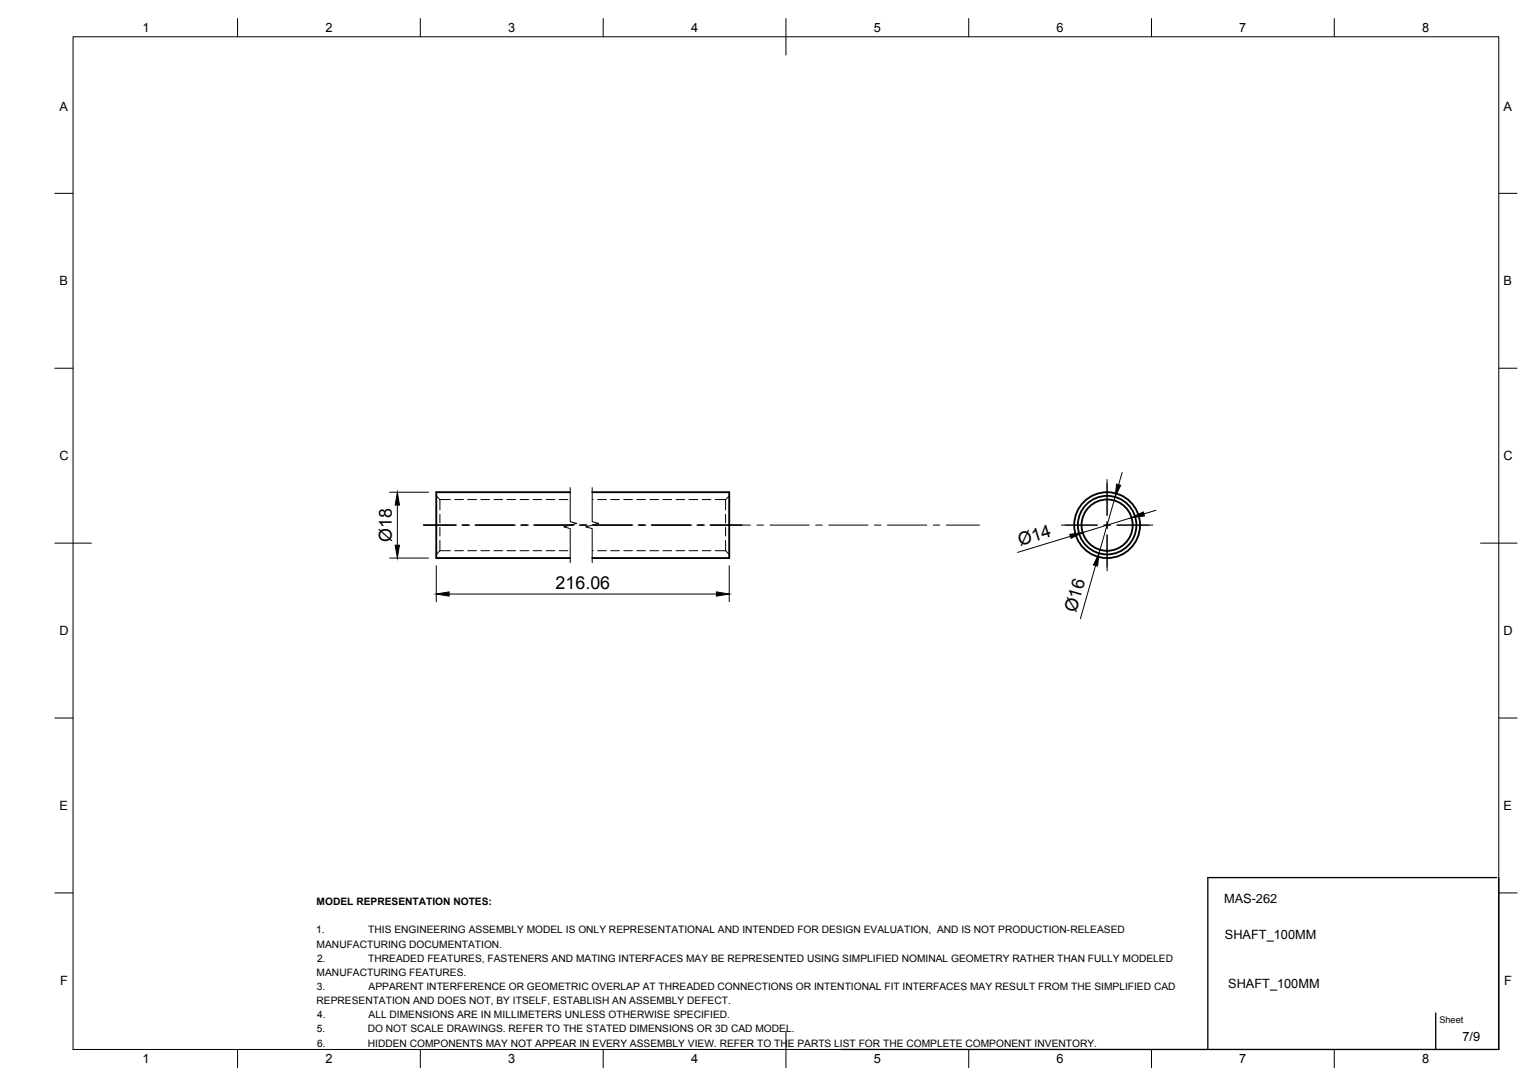
ISO-10303-21;
HEADER;
/* Generated by software containing ST-Developer
 * from STEP Tools, Inc. (www.steptools.com) 
 */

FILE_DESCRIPTION(
/* description */ (''),
/* implementation_level */ '2;1');

FILE_NAME(
/* name */ 'SHAFT_100MM.step',
/* time_stamp */ '2026-10-07T02:13:48+06:00',
/* author */ (''),
/* organization */ (''),
/* preprocessor_version */ 'ST-DEVELOPER v20.2',
/* originating_system */ 'Autodesk Translation Framework v15.15.0.0',
/* authorisation */ '');

FILE_SCHEMA (('AUTOMOTIVE_DESIGN { 1 0 10303 214 3 1 1 }'));
ENDSEC;

DATA;
#10=MECHANICAL_DESIGN_GEOMETRIC_PRESENTATION_REPRESENTATION('',(#118),#17042);
#59=CONICAL_SURFACE('',#8827,7.5,0.785398163397441);
#60=CONICAL_SURFACE('',#8834,7.5,0.785398163397441);
#94=SHAPE_REPRESENTATION_RELATIONSHIP('SRR','None',#17090,#106);
#106=ADVANCED_BREP_SHAPE_REPRESENTATION('',(#130),#17034);
#118=STYLED_ITEM('',(#17154),#130);
#130=MANIFOLD_SOLID_BREP('Body1',#8119);
#162=FACE_BOUND('',#1264,.T.);
#163=FACE_BOUND('',#1267,.T.);
#392=PLANE('',#8832);
#393=PLANE('',#8836);
#760=FACE_OUTER_BOUND('',#1261,.T.);
#761=FACE_OUTER_BOUND('',#1262,.T.);
#762=FACE_OUTER_BOUND('',#1263,.T.);
#763=FACE_OUTER_BOUND('',#1265,.T.);
#764=FACE_OUTER_BOUND('',#1266,.T.);
#765=FACE_OUTER_BOUND('',#1268,.T.);
#1261=EDGE_LOOP('',(#6519,#6520,#6521,#6522));
#1262=EDGE_LOOP('',(#6523,#6524,#6525,#6526));
#1263=EDGE_LOOP('',(#6527));
#1264=EDGE_LOOP('',(#6528));
#1265=EDGE_LOOP('',(#6529,#6530,#6531,#6532));
#1266=EDGE_LOOP('',(#6533));
#1267=EDGE_LOOP('',(#6534));
#1268=EDGE_LOOP('',(#6535,#6536,#6537,#6538));
#1764=CIRCLE('',#8828,8.);
#1765=CIRCLE('',#8829,7.);
#1766=CIRCLE('',#8831,7.);
#1767=CIRCLE('',#8833,9.);
#1768=CIRCLE('',#8835,8.);
#1769=CIRCLE('',#8837,9.);
#2426=LINE('',#13679,#3004);
#2427=LINE('',#13684,#3005);
#2428=LINE('',#13691,#3006);
#2429=LINE('',#13696,#3007);
#3004=VECTOR('',#10793,7.5);
#3005=VECTOR('',#10800,8.);
#3006=VECTOR('',#10809,7.5);
#3007=VECTOR('',#10816,9.);
#3619=VERTEX_POINT('',#13676);
#3620=VERTEX_POINT('',#13678);
#3621=VERTEX_POINT('',#13682);
#3622=VERTEX_POINT('',#13686);
#3623=VERTEX_POINT('',#13689);
#3624=VERTEX_POINT('',#13693);
#4627=EDGE_CURVE('',#3619,#3619,#1764,.T.);
#4628=EDGE_CURVE('',#3619,#3620,#2426,.T.);
#4629=EDGE_CURVE('',#3620,#3620,#1765,.T.);
#4630=EDGE_CURVE('',#3621,#3621,#1766,.T.);
#4631=EDGE_CURVE('',#3621,#3620,#2427,.T.);
#4632=EDGE_CURVE('',#3622,#3622,#1767,.T.);
#4633=EDGE_CURVE('',#3623,#3623,#1768,.T.);
#4634=EDGE_CURVE('',#3623,#3621,#2428,.T.);
#4635=EDGE_CURVE('',#3624,#3624,#1769,.T.);
#4636=EDGE_CURVE('',#3624,#3622,#2429,.T.);
#6519=ORIENTED_EDGE('',*,*,#4627,.T.);
#6520=ORIENTED_EDGE('',*,*,#4628,.T.);
#6521=ORIENTED_EDGE('',*,*,#4629,.T.);
#6522=ORIENTED_EDGE('',*,*,#4628,.F.);
#6523=ORIENTED_EDGE('',*,*,#4630,.F.);
#6524=ORIENTED_EDGE('',*,*,#4631,.T.);
#6525=ORIENTED_EDGE('',*,*,#4629,.F.);
#6526=ORIENTED_EDGE('',*,*,#4631,.F.);
#6527=ORIENTED_EDGE('',*,*,#4632,.T.);
#6528=ORIENTED_EDGE('',*,*,#4627,.F.);
#6529=ORIENTED_EDGE('',*,*,#4633,.T.);
#6530=ORIENTED_EDGE('',*,*,#4634,.T.);
#6531=ORIENTED_EDGE('',*,*,#4630,.T.);
#6532=ORIENTED_EDGE('',*,*,#4634,.F.);
#6533=ORIENTED_EDGE('',*,*,#4635,.T.);
#6534=ORIENTED_EDGE('',*,*,#4633,.F.);
#6535=ORIENTED_EDGE('',*,*,#4635,.F.);
#6536=ORIENTED_EDGE('',*,*,#4636,.T.);
#6537=ORIENTED_EDGE('',*,*,#4632,.F.);
#6538=ORIENTED_EDGE('',*,*,#4636,.F.);
#7569=CYLINDRICAL_SURFACE('',#8830,7.);
#7570=CYLINDRICAL_SURFACE('',#8838,9.);
#7922=ADVANCED_FACE('',(#760),#59,.F.);
#7923=ADVANCED_FACE('',(#761),#7569,.F.);
#7924=ADVANCED_FACE('',(#762,#162),#392,.T.);
#7925=ADVANCED_FACE('',(#763),#60,.F.);
#7926=ADVANCED_FACE('',(#764,#163),#393,.F.);
#7927=ADVANCED_FACE('',(#765),#7570,.T.);
#8119=CLOSED_SHELL('',(#7922,#7923,#7924,#7925,#7926,#7927));
#8826=AXIS2_PLACEMENT_3D('',#13674,#10787,#10788);
#8827=AXIS2_PLACEMENT_3D('',#13675,#10789,#10790);
#8828=AXIS2_PLACEMENT_3D('',#13677,#10791,#10792);
#8829=AXIS2_PLACEMENT_3D('',#13680,#10794,#10795);
#8830=AXIS2_PLACEMENT_3D('',#13681,#10796,#10797);
#8831=AXIS2_PLACEMENT_3D('',#13683,#10798,#10799);
#8832=AXIS2_PLACEMENT_3D('',#13685,#10801,#10802);
#8833=AXIS2_PLACEMENT_3D('',#13687,#10803,#10804);
#8834=AXIS2_PLACEMENT_3D('',#13688,#10805,#10806);
#8835=AXIS2_PLACEMENT_3D('',#13690,#10807,#10808);
#8836=AXIS2_PLACEMENT_3D('',#13692,#10810,#10811);
#8837=AXIS2_PLACEMENT_3D('',#13694,#10812,#10813);
#8838=AXIS2_PLACEMENT_3D('',#13695,#10814,#10815);
#10787=DIRECTION('axis',(0.,0.,1.));
#10788=DIRECTION('refdir',(1.,0.,0.));
#10789=DIRECTION('center_axis',(0.,0.,-1.));
#10790=DIRECTION('ref_axis',(-1.,0.,0.));
#10791=DIRECTION('center_axis',(0.,0.,-1.));
#10792=DIRECTION('ref_axis',(-1.,0.,0.));
#10793=DIRECTION('',(-0.707106781186542,8.65956056235487E-17,0.707106781186553));
#10794=DIRECTION('center_axis',(0.,0.,1.));
#10795=DIRECTION('ref_axis',(-1.,0.,0.));
#10796=DIRECTION('center_axis',(0.,0.,1.));
#10797=DIRECTION('ref_axis',(-1.,0.,0.));
#10798=DIRECTION('center_axis',(0.,0.,-1.));
#10799=DIRECTION('ref_axis',(-1.,0.,0.));
#10800=DIRECTION('',(0.,0.,-1.));
#10801=DIRECTION('center_axis',(0.,0.,-1.));
#10802=DIRECTION('ref_axis',(-1.,0.,0.));
#10803=DIRECTION('center_axis',(0.,0.,-1.));
#10804=DIRECTION('ref_axis',(-1.,0.,0.));
#10805=DIRECTION('center_axis',(0.,0.,1.));
#10806=DIRECTION('ref_axis',(-1.,0.,0.));
#10807=DIRECTION('center_axis',(0.,0.,1.));
#10808=DIRECTION('ref_axis',(-1.,0.,0.));
#10809=DIRECTION('',(-0.707106781186542,-8.65956056235487E-17,-0.707106781186553));
#10810=DIRECTION('center_axis',(0.,0.,-1.));
#10811=DIRECTION('ref_axis',(-1.,0.,0.));
#10812=DIRECTION('center_axis',(0.,0.,1.));
#10813=DIRECTION('ref_axis',(-1.,0.,0.));
#10814=DIRECTION('center_axis',(0.,0.,1.));
#10815=DIRECTION('ref_axis',(-1.,0.,0.));
#10816=DIRECTION('',(0.,0.,-1.));
#13674=CARTESIAN_POINT('',(0.,0.,0.));
#13675=CARTESIAN_POINT('Origin',(-6.5,6.43177298256785,247.386209595194));
#13676=CARTESIAN_POINT('',(1.5,6.43177298256785,246.886209595194));
#13677=CARTESIAN_POINT('Origin',(-6.5,6.43177298256785,246.886209595194));
#13678=CARTESIAN_POINT('',(0.499999999999999,6.43177298256785,247.886209595194));
#13679=CARTESIAN_POINT('',(0.999999999999999,6.43177298256785,247.386209595194));
#13680=CARTESIAN_POINT('Origin',(-6.5,6.43177298256785,247.886209595194));
#13681=CARTESIAN_POINT('Origin',(-6.5,6.43177298256785,246.886209595194));
#13682=CARTESIAN_POINT('',(0.499999999999999,6.43177298256785,461.946209595194));
#13683=CARTESIAN_POINT('Origin',(-6.5,6.43177298256785,461.946209595194));
#13684=CARTESIAN_POINT('',(0.499999999999999,6.43177298256785,246.886209595194));
#13685=CARTESIAN_POINT('Origin',(-6.5,6.43177298256785,246.886209595194));
#13686=CARTESIAN_POINT('',(2.5,6.43177298256785,246.886209595194));
#13687=CARTESIAN_POINT('Origin',(-6.5,6.43177298256785,246.886209595194));
#13688=CARTESIAN_POINT('Origin',(-6.5,6.43177298256785,462.446209595194));
#13689=CARTESIAN_POINT('',(1.5,6.43177298256785,462.946209595194));
#13690=CARTESIAN_POINT('Origin',(-6.5,6.43177298256785,462.946209595194));
#13691=CARTESIAN_POINT('',(0.999999999999999,6.43177298256785,462.446209595194));
#13692=CARTESIAN_POINT('Origin',(-6.5,6.43177298256785,462.946209595194));
#13693=CARTESIAN_POINT('',(2.5,6.43177298256785,462.946209595194));
#13694=CARTESIAN_POINT('Origin',(-6.5,6.43177298256785,462.946209595194));
#13695=CARTESIAN_POINT('Origin',(-6.5,6.43177298256785,246.886209595194));
#13696=CARTESIAN_POINT('',(2.5,6.43177298256785,246.886209595194));
#17020=UNCERTAINTY_MEASURE_WITH_UNIT(LENGTH_MEASURE(0.01),#17043,
'DISTANCE_ACCURACY_VALUE',
'Maximum model space distance between geometric entities at asserted c
onnectivities');
#17028=UNCERTAINTY_MEASURE_WITH_UNIT(LENGTH_MEASURE(0.01),#17043,
'DISTANCE_ACCURACY_VALUE',
'Maximum model space distance between geometric entities at asserted c
onnectivities');
#17034=(
GEOMETRIC_REPRESENTATION_CONTEXT(3)
GLOBAL_UNCERTAINTY_ASSIGNED_CONTEXT((#17020))
GLOBAL_UNIT_ASSIGNED_CONTEXT((#17043,#17045,#17046))
REPRESENTATION_CONTEXT('','3D')
);
#17042=(
GEOMETRIC_REPRESENTATION_CONTEXT(3)
GLOBAL_UNCERTAINTY_ASSIGNED_CONTEXT((#17028))
GLOBAL_UNIT_ASSIGNED_CONTEXT((#17043,#17045,#17046))
REPRESENTATION_CONTEXT('','3D')
);
#17043=(
LENGTH_UNIT()
NAMED_UNIT(*)
SI_UNIT(.MILLI.,.METRE.)
);
#17045=(
NAMED_UNIT(*)
PLANE_ANGLE_UNIT()
SI_UNIT($,.RADIAN.)
);
#17046=(
NAMED_UNIT(*)
SI_UNIT($,.STERADIAN.)
SOLID_ANGLE_UNIT()
);
#17052=SHAPE_DEFINITION_REPRESENTATION(#17065,#17090);
#17065=PRODUCT_DEFINITION_SHAPE('',$,#17104);
#17090=SHAPE_REPRESENTATION('',(#8826),#17034);
#17098=PRODUCT_DEFINITION_CONTEXT('part definition',#17139,'design');
#17104=PRODUCT_DEFINITION('SHAFT_100MM','SHAFT_100MM',#17117,#17098);
#17117=PRODUCT_DEFINITION_FORMATION('',$,#17146);
#17139=APPLICATION_CONTEXT(
'Core Data for Automotive Mechanical Design Process');
#17140=PRODUCT_CONTEXT('part definition',#17139,'mechanical');
#17146=PRODUCT('SHAFT_100MM','SHAFT_100MM',$,(#17140));
#17154=PRESENTATION_STYLE_ASSIGNMENT((#17155));
#17155=SURFACE_STYLE_USAGE(.BOTH.,#17156);
#17156=SURFACE_SIDE_STYLE('',(#17157));
#17157=SURFACE_STYLE_FILL_AREA(#17158);
#17158=FILL_AREA_STYLE('Steel - Satin',(#17159));
#17159=FILL_AREA_STYLE_COLOUR('Steel - Satin',#17160);
#17160=COLOUR_RGB('Steel - Satin', 0.09019608, 0.27058824, 0.51372549);
ENDSEC;
END-ISO-10303-21;
